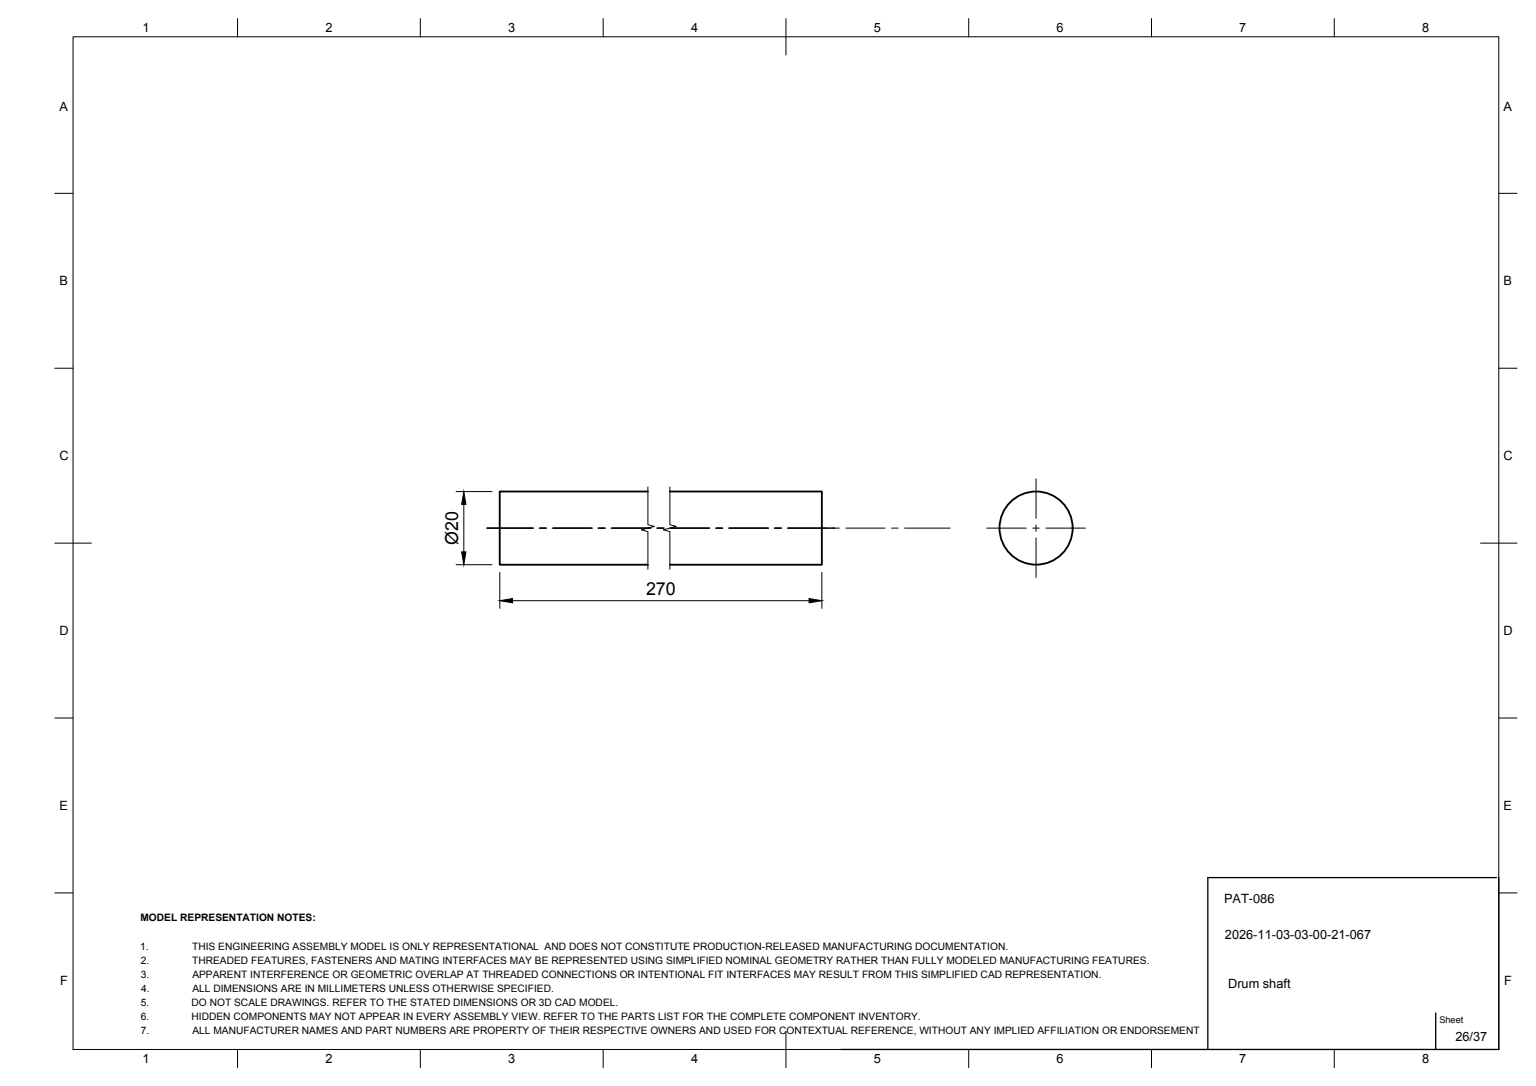
ISO-10303-21;
HEADER;
/* Generated by software containing ST-Developer
 * from STEP Tools, Inc. (www.steptools.com) 
 */

FILE_DESCRIPTION(
/* description */ ('Ratchet and pawl hand winch drum'),
/* implementation_level */ '2;1');

FILE_NAME(
/* name */ 'Drum shaft.step',
/* time_stamp */ '2026-10-27T12:42:58-07:00',
/* author */ (''),
/* organization */ (''),
/* preprocessor_version */ 'ST-DEVELOPER v20.2',
/* originating_system */ 'Autodesk Translation Framework v15.17.0.0',
/* authorisation */ '');

FILE_SCHEMA (('AUTOMOTIVE_DESIGN { 1 0 10303 214 3 1 1 }'));
ENDSEC;

DATA;
#10=MECHANICAL_DESIGN_GEOMETRIC_PRESENTATION_REPRESENTATION('',(#410),#11801);
#341=SHAPE_REPRESENTATION_RELATIONSHIP('SRR','None',#11969,#375);
#375=ADVANCED_BREP_SHAPE_REPRESENTATION('',(#443),#11786);
#410=STYLED_ITEM('',(#12213),#443);
#443=MANIFOLD_SOLID_BREP('Body1',#6289);
#726=PLANE('',#7054);
#727=PLANE('',#7055);
#1043=FACE_OUTER_BOUND('',#1507,.T.);
#1044=FACE_OUTER_BOUND('',#1508,.T.);
#1045=FACE_OUTER_BOUND('',#1509,.T.);
#1507=EDGE_LOOP('',(#5101,#5102,#5103,#5104));
#1508=EDGE_LOOP('',(#5105));
#1509=EDGE_LOOP('',(#5106));
#1958=LINE('',#10586,#2469);
#2469=VECTOR('',#8367,1.);
#2861=CIRCLE('',#7052,1.);
#2862=CIRCLE('',#7053,1.);
#3232=VERTEX_POINT('',#10583);
#3233=VERTEX_POINT('',#10585);
#3894=EDGE_CURVE('',#3232,#3232,#2861,.T.);
#3895=EDGE_CURVE('',#3232,#3233,#1958,.T.);
#3896=EDGE_CURVE('',#3233,#3233,#2862,.T.);
#5101=ORIENTED_EDGE('',*,*,#3894,.F.);
#5102=ORIENTED_EDGE('',*,*,#3895,.T.);
#5103=ORIENTED_EDGE('',*,*,#3896,.T.);
#5104=ORIENTED_EDGE('',*,*,#3895,.F.);
#5105=ORIENTED_EDGE('',*,*,#3894,.T.);
#5106=ORIENTED_EDGE('',*,*,#3896,.F.);
#5877=CYLINDRICAL_SURFACE('',#7051,1.);
#6113=ADVANCED_FACE('',(#1043),#5877,.T.);
#6114=ADVANCED_FACE('',(#1044),#726,.T.);
#6115=ADVANCED_FACE('',(#1045),#727,.F.);
#6289=CLOSED_SHELL('',(#6113,#6114,#6115));
#7050=AXIS2_PLACEMENT_3D('',#10581,#8361,#8362);
#7051=AXIS2_PLACEMENT_3D('',#10582,#8363,#8364);
#7052=AXIS2_PLACEMENT_3D('',#10584,#8365,#8366);
#7053=AXIS2_PLACEMENT_3D('',#10587,#8368,#8369);
#7054=AXIS2_PLACEMENT_3D('',#10588,#8370,#8371);
#7055=AXIS2_PLACEMENT_3D('',#10589,#8372,#8373);
#8361=DIRECTION('axis',(0.,0.,1.));
#8362=DIRECTION('refdir',(1.,0.,0.));
#8363=DIRECTION('center_axis',(0.,1.,0.));
#8364=DIRECTION('ref_axis',(1.,0.,0.));
#8365=DIRECTION('center_axis',(0.,1.,0.));
#8366=DIRECTION('ref_axis',(1.,0.,0.));
#8367=DIRECTION('',(0.,-1.,0.));
#8368=DIRECTION('center_axis',(0.,1.,0.));
#8369=DIRECTION('ref_axis',(1.,0.,0.));
#8370=DIRECTION('center_axis',(0.,1.,0.));
#8371=DIRECTION('ref_axis',(1.,0.,0.));
#8372=DIRECTION('center_axis',(0.,1.,0.));
#8373=DIRECTION('ref_axis',(1.,0.,0.));
#10581=CARTESIAN_POINT('',(0.,0.,0.));
#10582=CARTESIAN_POINT('Origin',(0.,-7.,6.53));
#10583=CARTESIAN_POINT('',(-1.,20.,6.53));
#10584=CARTESIAN_POINT('Origin',(0.,20.,6.53));
#10585=CARTESIAN_POINT('',(-1.,-7.,6.53));
#10586=CARTESIAN_POINT('',(-1.,-7.,6.53));
#10587=CARTESIAN_POINT('Origin',(0.,-7.,6.53));
#10588=CARTESIAN_POINT('Origin',(0.,20.,6.53));
#10589=CARTESIAN_POINT('Origin',(0.,-7.,6.53));
#11746=UNCERTAINTY_MEASURE_WITH_UNIT(LENGTH_MEASURE(0.001),#11802,
'DISTANCE_ACCURACY_VALUE',
'Maximum model space distance between geometric entities at asserted c
onnectivities');
#11761=UNCERTAINTY_MEASURE_WITH_UNIT(LENGTH_MEASURE(0.001),#11802,
'DISTANCE_ACCURACY_VALUE',
'Maximum model space distance between geometric entities at asserted c
onnectivities');
#11786=(
GEOMETRIC_REPRESENTATION_CONTEXT(3)
GLOBAL_UNCERTAINTY_ASSIGNED_CONTEXT((#11746))
GLOBAL_UNIT_ASSIGNED_CONTEXT((#11802,#11804,#11805))
REPRESENTATION_CONTEXT('','3D')
);
#11801=(
GEOMETRIC_REPRESENTATION_CONTEXT(3)
GLOBAL_UNCERTAINTY_ASSIGNED_CONTEXT((#11761))
GLOBAL_UNIT_ASSIGNED_CONTEXT((#11802,#11804,#11805))
REPRESENTATION_CONTEXT('','3D')
);
#11802=(
LENGTH_UNIT()
NAMED_UNIT(*)
SI_UNIT(.CENTI.,.METRE.)
);
#11804=(
NAMED_UNIT(*)
PLANE_ANGLE_UNIT()
SI_UNIT($,.RADIAN.)
);
#11805=(
NAMED_UNIT(*)
SI_UNIT($,.STERADIAN.)
SOLID_ANGLE_UNIT()
);
#11830=SHAPE_DEFINITION_REPRESENTATION(#11871,#11969);
#11871=PRODUCT_DEFINITION_SHAPE('',$,#12009);
#11969=SHAPE_REPRESENTATION('',(#7050),#11786);
#11984=PRODUCT_DEFINITION_CONTEXT('part definition',#12103,'design');
#12009=PRODUCT_DEFINITION('Drum shaft','Drum shaft',#12048,#11984);
#12048=PRODUCT_DEFINITION_FORMATION('',$,#12129);
#12103=APPLICATION_CONTEXT(
'Core Data for Automotive Mechanical Design Process');
#12104=PRODUCT_CONTEXT('part definition',#12103,'mechanical');
#12129=PRODUCT('Drum shaft','Drum shaft','Drum shaft',(#12104));
#12207=COLOUR_RGB('Grey',0.48,0.52,0.57);
#12208=FILL_AREA_STYLE_COLOUR('',#12207);
#12209=FILL_AREA_STYLE('',(#12208));
#12210=SURFACE_STYLE_FILL_AREA(#12209);
#12211=SURFACE_SIDE_STYLE('',(#12210));
#12212=SURFACE_STYLE_USAGE(.BOTH.,#12211);
#12213=PRESENTATION_STYLE_ASSIGNMENT((#12212));
ENDSEC;
END-ISO-10303-21;
